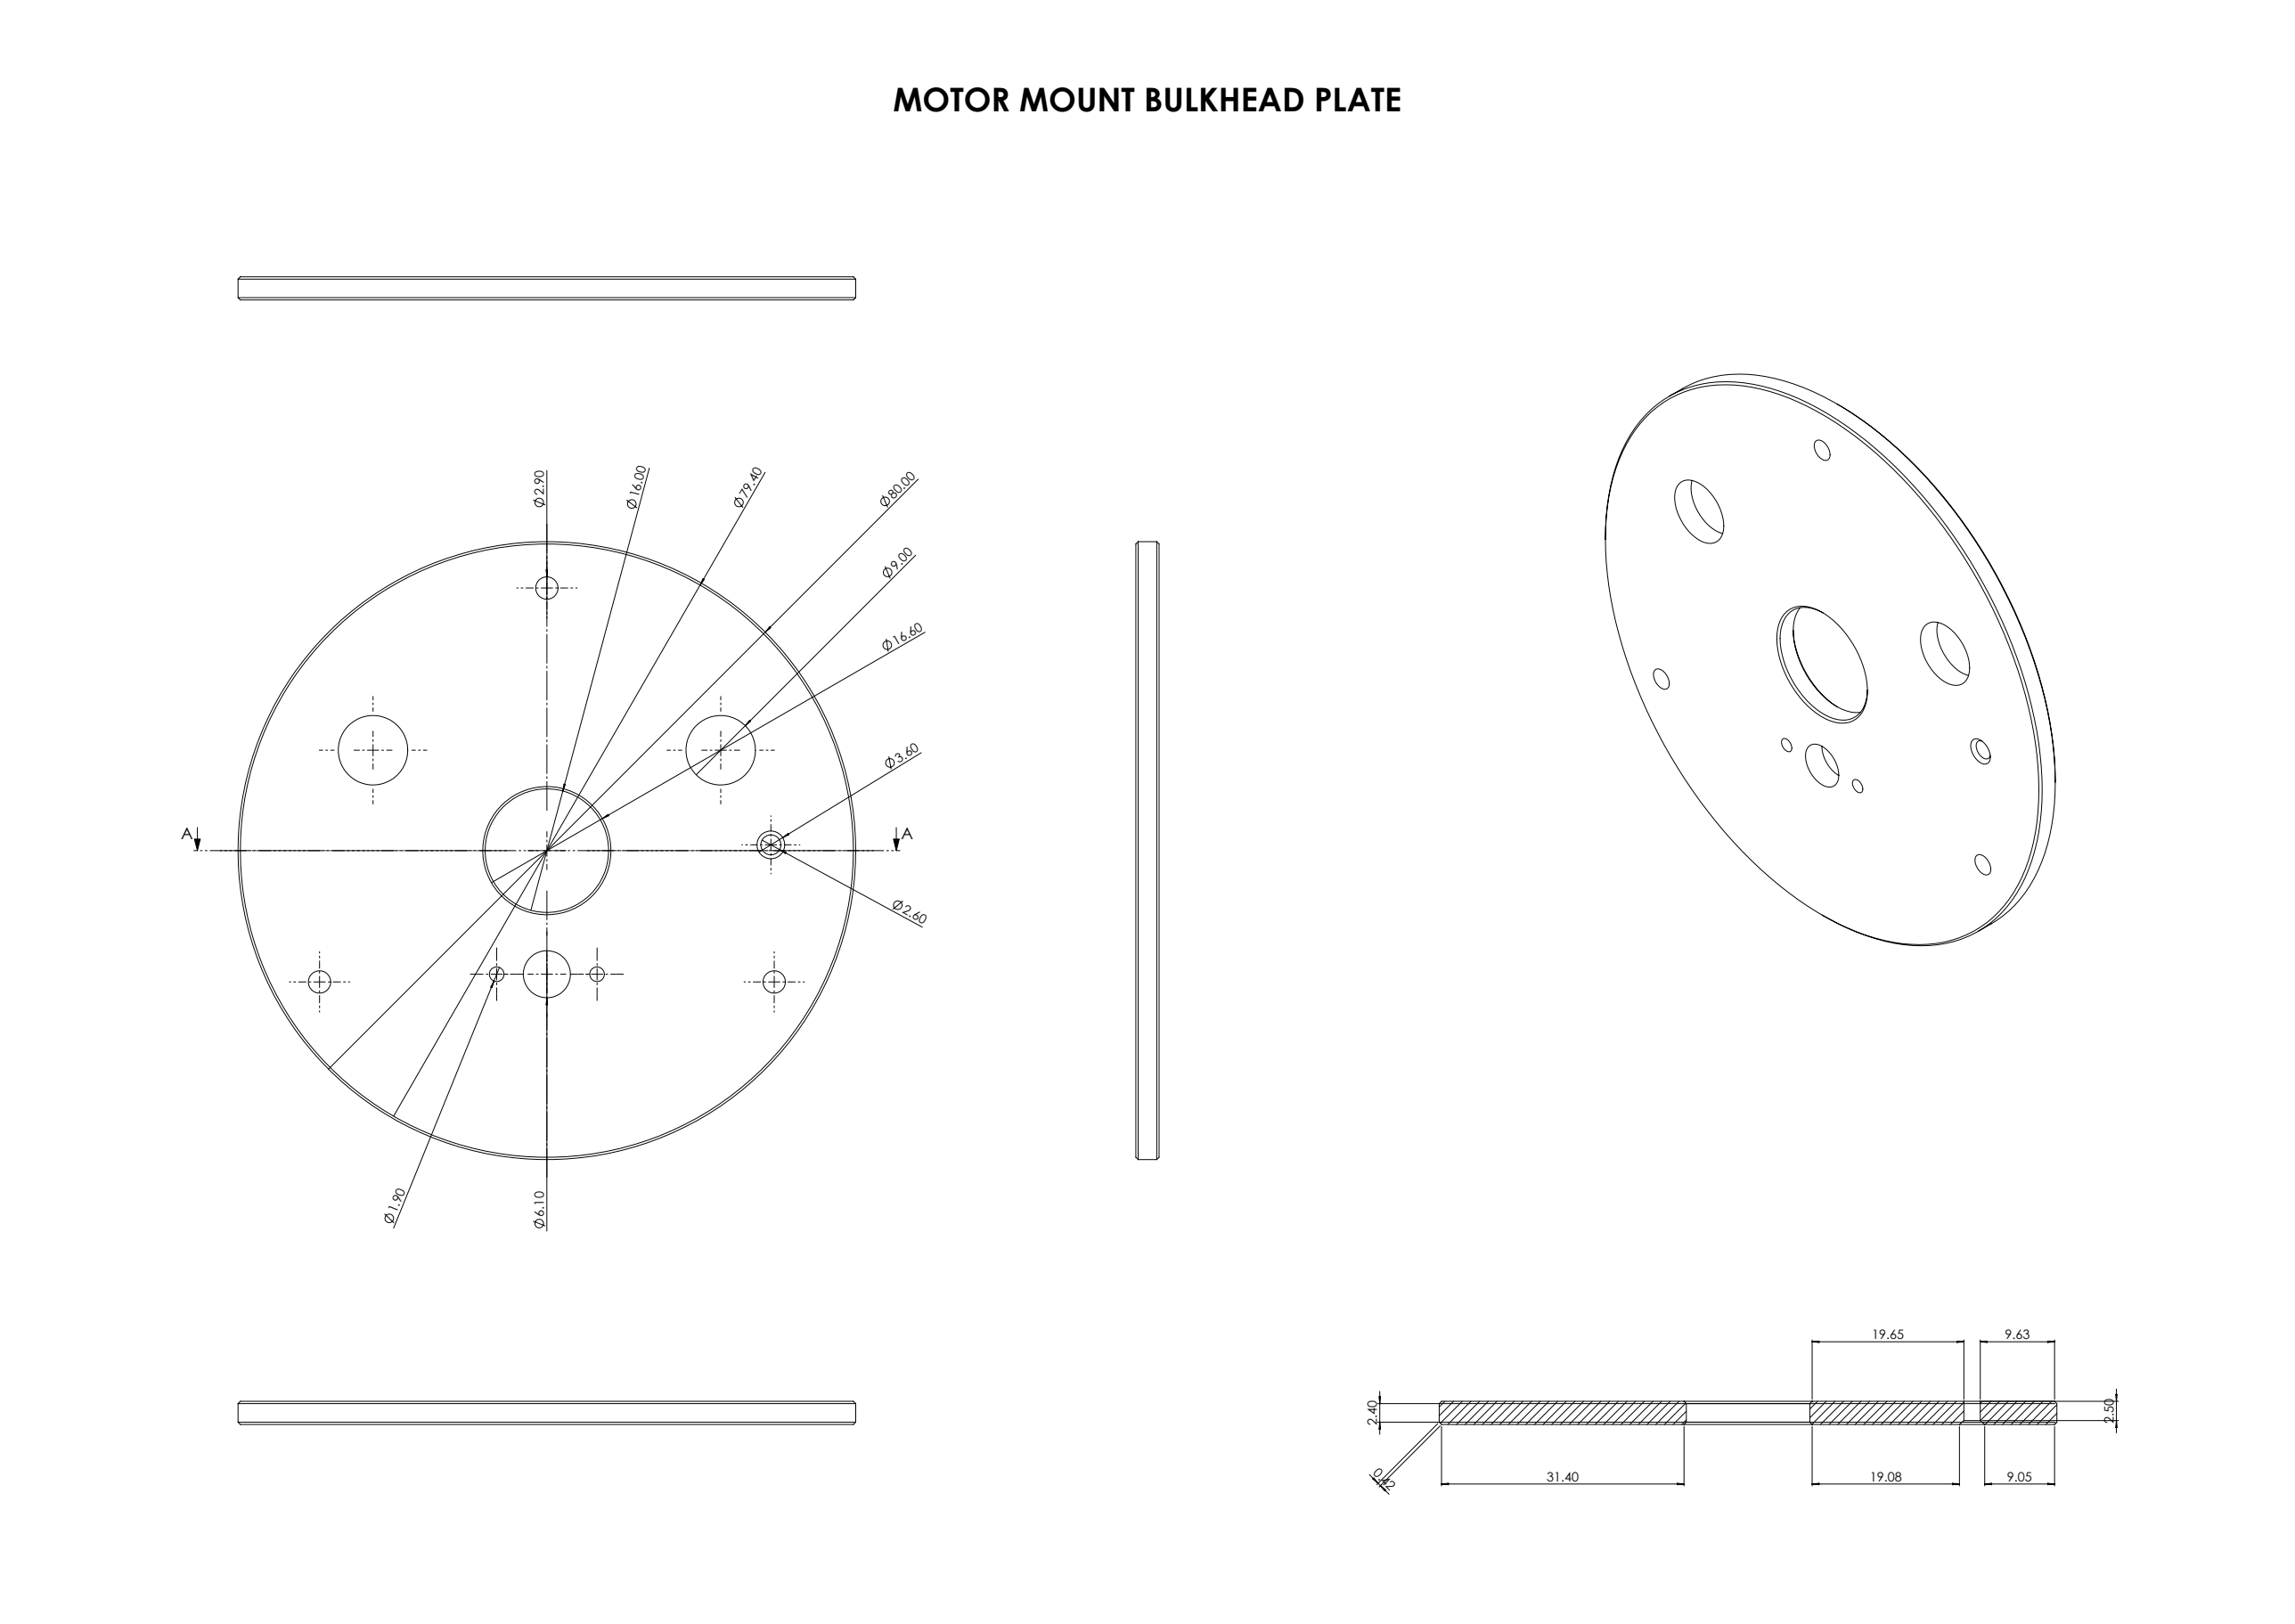
ISO-10303-21;
HEADER;
/* Generated by software containing ST-Developer
 * from STEP Tools, Inc. (www.steptools.com) 
 */

FILE_DESCRIPTION(
/* description */ (''),
/* implementation_level */ '2;1');

FILE_NAME(
/* name */ '06_Motor_Mount_Bulkhead_Plate.step',
/* time_stamp */ '2026-10-19T23:00:43-07:00',
/* author */ (''),
/* organization */ (''),
/* preprocessor_version */ 'ST-DEVELOPER v20.2',
/* originating_system */ 'Autodesk Translation Framework v15.15.0.0',
/* authorisation */ '');

FILE_SCHEMA (('AUTOMOTIVE_DESIGN { 1 0 10303 214 3 1 1 }'));
ENDSEC;

DATA;
#10=MECHANICAL_DESIGN_GEOMETRIC_PRESENTATION_REPRESENTATION('',(#1001),#55002);
#961=SHAPE_REPRESENTATION_RELATIONSHIP('SRR','None',#55109,#981);
#981=ADVANCED_BREP_SHAPE_REPRESENTATION('',(#1021),#54987);
#1001=STYLED_ITEM('',(#55372),#1021);
#1021=MANIFOLD_SOLID_BREP('Motor Mount Bulkhead',#24534);
#1169=FACE_BOUND('',#4389,.T.);
#1170=FACE_BOUND('',#4390,.T.);
#1171=FACE_BOUND('',#4391,.T.);
#1172=FACE_BOUND('',#4392,.T.);
#1173=FACE_BOUND('',#4393,.T.);
#1174=FACE_BOUND('',#4394,.T.);
#1175=FACE_BOUND('',#4395,.T.);
#1176=FACE_BOUND('',#4396,.T.);
#1177=FACE_BOUND('',#4397,.T.);
#1178=FACE_BOUND('',#4398,.T.);
#1179=FACE_BOUND('',#4401,.T.);
#1180=FACE_BOUND('',#4402,.T.);
#1181=FACE_BOUND('',#4403,.T.);
#1182=FACE_BOUND('',#4404,.T.);
#1183=FACE_BOUND('',#4405,.T.);
#1184=FACE_BOUND('',#4406,.T.);
#1185=FACE_BOUND('',#4407,.T.);
#1186=FACE_BOUND('',#4408,.T.);
#1187=FACE_BOUND('',#4409,.T.);
#1188=FACE_BOUND('',#4410,.T.);
#1423=PLANE('',#25786);
#1424=PLANE('',#25790);
#2128=CYLINDRICAL_SURFACE('',#25750,0.45);
#2129=CYLINDRICAL_SURFACE('',#25753,0.45);
#2130=CYLINDRICAL_SURFACE('',#25756,0.13);
#2131=CYLINDRICAL_SURFACE('',#25761,0.145);
#2132=CYLINDRICAL_SURFACE('',#25764,0.145);
#2133=CYLINDRICAL_SURFACE('',#25767,0.145);
#2134=CYLINDRICAL_SURFACE('',#25770,0.0950000000000001);
#2135=CYLINDRICAL_SURFACE('',#25773,0.095);
#2136=CYLINDRICAL_SURFACE('',#25776,0.305);
#2137=CYLINDRICAL_SURFACE('',#25783,0.8);
#2138=CYLINDRICAL_SURFACE('',#25795,4.);
#2879=FACE_OUTER_BOUND('',#4376,.T.);
#2880=FACE_OUTER_BOUND('',#4377,.T.);
#2881=FACE_OUTER_BOUND('',#4378,.T.);
#2882=FACE_OUTER_BOUND('',#4379,.T.);
#2883=FACE_OUTER_BOUND('',#4380,.T.);
#2884=FACE_OUTER_BOUND('',#4381,.T.);
#2885=FACE_OUTER_BOUND('',#4382,.T.);
#2886=FACE_OUTER_BOUND('',#4383,.T.);
#2887=FACE_OUTER_BOUND('',#4384,.T.);
#2888=FACE_OUTER_BOUND('',#4385,.T.);
#2889=FACE_OUTER_BOUND('',#4386,.T.);
#2890=FACE_OUTER_BOUND('',#4387,.T.);
#2891=FACE_OUTER_BOUND('',#4388,.T.);
#2892=FACE_OUTER_BOUND('',#4399,.T.);
#2893=FACE_OUTER_BOUND('',#4400,.T.);
#2894=FACE_OUTER_BOUND('',#4411,.T.);
#2895=FACE_OUTER_BOUND('',#4412,.T.);
#2896=FACE_OUTER_BOUND('',#4413,.T.);
#4376=EDGE_LOOP('',(#18006,#18007,#18008,#18009));
#4377=EDGE_LOOP('',(#18010,#18011,#18012,#18013));
#4378=EDGE_LOOP('',(#18014,#18015,#18016,#18017));
#4379=EDGE_LOOP('',(#18018,#18019,#18020,#18021));
#4380=EDGE_LOOP('',(#18022,#18023,#18024,#18025));
#4381=EDGE_LOOP('',(#18026,#18027,#18028,#18029));
#4382=EDGE_LOOP('',(#18030,#18031,#18032,#18033));
#4383=EDGE_LOOP('',(#18034,#18035,#18036,#18037));
#4384=EDGE_LOOP('',(#18038,#18039,#18040,#18041));
#4385=EDGE_LOOP('',(#18042,#18043,#18044,#18045));
#4386=EDGE_LOOP('',(#18046,#18047,#18048,#18049,#18050));
#4387=EDGE_LOOP('',(#18051,#18052,#18053,#18054,#18055,#18056));
#4388=EDGE_LOOP('',(#18057));
#4389=EDGE_LOOP('',(#18058));
#4390=EDGE_LOOP('',(#18059));
#4391=EDGE_LOOP('',(#18060));
#4392=EDGE_LOOP('',(#18061));
#4393=EDGE_LOOP('',(#18062));
#4394=EDGE_LOOP('',(#18063));
#4395=EDGE_LOOP('',(#18064));
#4396=EDGE_LOOP('',(#18065));
#4397=EDGE_LOOP('',(#18066));
#4398=EDGE_LOOP('',(#18067));
#4399=EDGE_LOOP('',(#18068,#18069,#18070,#18071,#18072));
#4400=EDGE_LOOP('',(#18073));
#4401=EDGE_LOOP('',(#18074));
#4402=EDGE_LOOP('',(#18075));
#4403=EDGE_LOOP('',(#18076));
#4404=EDGE_LOOP('',(#18077));
#4405=EDGE_LOOP('',(#18078));
#4406=EDGE_LOOP('',(#18079));
#4407=EDGE_LOOP('',(#18080));
#4408=EDGE_LOOP('',(#18081));
#4409=EDGE_LOOP('',(#18082));
#4410=EDGE_LOOP('',(#18083));
#4411=EDGE_LOOP('',(#18084,#18085,#18086,#18087,#18088));
#4412=EDGE_LOOP('',(#18089,#18090,#18091,#18092,#18093,#18094));
#4413=EDGE_LOOP('',(#18095,#18096,#18097,#18098,#18099));
#5932=LINE('',#36111,#7753);
#5933=LINE('',#36117,#7754);
#5934=LINE('',#36123,#7755);
#5935=LINE('',#36127,#7756);
#5936=LINE('',#36133,#7757);
#5937=LINE('',#36139,#7758);
#5938=LINE('',#36145,#7759);
#5939=LINE('',#36151,#7760);
#5940=LINE('',#36157,#7761);
#5941=LINE('',#36163,#7762);
#5942=LINE('',#36169,#7763);
#5943=LINE('',#36178,#7764);
#5944=LINE('',#36184,#7765);
#5945=LINE('',#36191,#7766);
#5946=LINE('',#36197,#7767);
#5947=LINE('',#36202,#7768);
#7753=VECTOR('',#29712,0.45);
#7754=VECTOR('',#29719,0.45);
#7755=VECTOR('',#29726,0.13);
#7756=VECTOR('',#29731,0.18);
#7757=VECTOR('',#29738,0.145);
#7758=VECTOR('',#29745,0.145);
#7759=VECTOR('',#29752,0.145);
#7760=VECTOR('',#29759,0.0950000000000001);
#7761=VECTOR('',#29766,0.095);
#7762=VECTOR('',#29773,0.305);
#7763=VECTOR('',#29780,0.815);
#7764=VECTOR('',#29791,0.8);
#7765=VECTOR('',#29798,0.815);
#7766=VECTOR('',#29807,3.985);
#7767=VECTOR('',#29814,4.);
#7768=VECTOR('',#29821,3.985);
#9528=CIRCLE('',#25751,0.45);
#9529=CIRCLE('',#25752,0.45);
#9530=CIRCLE('',#25754,0.45);
#9531=CIRCLE('',#25755,0.45);
#9532=CIRCLE('',#25757,0.13);
#9533=CIRCLE('',#25758,0.13);
#9534=CIRCLE('',#25760,0.18);
#9535=CIRCLE('',#25762,0.145);
#9536=CIRCLE('',#25763,0.145);
#9537=CIRCLE('',#25765,0.145);
#9538=CIRCLE('',#25766,0.145);
#9539=CIRCLE('',#25768,0.145);
#9540=CIRCLE('',#25769,0.145);
#9541=CIRCLE('',#25771,0.0950000000000001);
#9542=CIRCLE('',#25772,0.0950000000000001);
#9543=CIRCLE('',#25774,0.095);
#9544=CIRCLE('',#25775,0.095);
#9545=CIRCLE('',#25777,0.305);
#9546=CIRCLE('',#25778,0.305);
#9547=CIRCLE('',#25780,0.83);
#9548=CIRCLE('',#25781,0.8);
#9549=CIRCLE('',#25782,0.8);
#9550=CIRCLE('',#25784,0.8);
#9551=CIRCLE('',#25785,0.8);
#9552=CIRCLE('',#25787,3.97);
#9553=CIRCLE('',#25789,0.83);
#9554=CIRCLE('',#25791,3.97);
#9555=CIRCLE('',#25793,4.);
#9556=CIRCLE('',#25794,4.);
#9557=CIRCLE('',#25796,4.);
#9558=CIRCLE('',#25797,4.);
#10712=VERTEX_POINT('',#36108);
#10713=VERTEX_POINT('',#36110);
#10714=VERTEX_POINT('',#36114);
#10715=VERTEX_POINT('',#36116);
#10716=VERTEX_POINT('',#36120);
#10717=VERTEX_POINT('',#36122);
#10718=VERTEX_POINT('',#36126);
#10719=VERTEX_POINT('',#36130);
#10720=VERTEX_POINT('',#36132);
#10721=VERTEX_POINT('',#36136);
#10722=VERTEX_POINT('',#36138);
#10723=VERTEX_POINT('',#36142);
#10724=VERTEX_POINT('',#36144);
#10725=VERTEX_POINT('',#36148);
#10726=VERTEX_POINT('',#36150);
#10727=VERTEX_POINT('',#36154);
#10728=VERTEX_POINT('',#36156);
#10729=VERTEX_POINT('',#36160);
#10730=VERTEX_POINT('',#36162);
#10731=VERTEX_POINT('',#36166);
#10732=VERTEX_POINT('',#36168);
#10733=VERTEX_POINT('',#36170);
#10734=VERTEX_POINT('',#36174);
#10735=VERTEX_POINT('',#36175);
#10736=VERTEX_POINT('',#36180);
#10737=VERTEX_POINT('',#36183);
#10738=VERTEX_POINT('',#36187);
#10739=VERTEX_POINT('',#36190);
#10740=VERTEX_POINT('',#36192);
#10741=VERTEX_POINT('',#36196);
#10742=VERTEX_POINT('',#36198);
#13411=EDGE_CURVE('',#10712,#10712,#9528,.T.);
#13412=EDGE_CURVE('',#10712,#10713,#5932,.T.);
#13413=EDGE_CURVE('',#10713,#10713,#9529,.T.);
#13414=EDGE_CURVE('',#10714,#10714,#9530,.T.);
#13415=EDGE_CURVE('',#10714,#10715,#5933,.T.);
#13416=EDGE_CURVE('',#10715,#10715,#9531,.T.);
#13417=EDGE_CURVE('',#10716,#10716,#9532,.T.);
#13418=EDGE_CURVE('',#10716,#10717,#5934,.T.);
#13419=EDGE_CURVE('',#10717,#10717,#9533,.T.);
#13420=EDGE_CURVE('',#10717,#10718,#5935,.T.);
#13421=EDGE_CURVE('',#10718,#10718,#9534,.T.);
#13422=EDGE_CURVE('',#10719,#10719,#9535,.T.);
#13423=EDGE_CURVE('',#10719,#10720,#5936,.T.);
#13424=EDGE_CURVE('',#10720,#10720,#9536,.T.);
#13425=EDGE_CURVE('',#10721,#10721,#9537,.T.);
#13426=EDGE_CURVE('',#10721,#10722,#5937,.T.);
#13427=EDGE_CURVE('',#10722,#10722,#9538,.T.);
#13428=EDGE_CURVE('',#10723,#10723,#9539,.T.);
#13429=EDGE_CURVE('',#10723,#10724,#5938,.T.);
#13430=EDGE_CURVE('',#10724,#10724,#9540,.T.);
#13431=EDGE_CURVE('',#10725,#10725,#9541,.T.);
#13432=EDGE_CURVE('',#10725,#10726,#5939,.T.);
#13433=EDGE_CURVE('',#10726,#10726,#9542,.T.);
#13434=EDGE_CURVE('',#10727,#10727,#9543,.T.);
#13435=EDGE_CURVE('',#10727,#10728,#5940,.T.);
#13436=EDGE_CURVE('',#10728,#10728,#9544,.T.);
#13437=EDGE_CURVE('',#10729,#10729,#9545,.T.);
#13438=EDGE_CURVE('',#10729,#10730,#5941,.T.);
#13439=EDGE_CURVE('',#10730,#10730,#9546,.T.);
#13440=EDGE_CURVE('',#10731,#10731,#9547,.T.);
#13441=EDGE_CURVE('',#10731,#10732,#5942,.T.);
#13442=EDGE_CURVE('',#10732,#10733,#9548,.T.);
#13443=EDGE_CURVE('',#10733,#10732,#9549,.T.);
#13444=EDGE_CURVE('',#10734,#10735,#9550,.T.);
#13445=EDGE_CURVE('',#10735,#10734,#9551,.T.);
#13446=EDGE_CURVE('',#10735,#10733,#5943,.T.);
#13447=EDGE_CURVE('',#10736,#10736,#9552,.T.);
#13448=EDGE_CURVE('',#10734,#10737,#5944,.T.);
#13449=EDGE_CURVE('',#10737,#10737,#9553,.T.);
#13450=EDGE_CURVE('',#10738,#10738,#9554,.T.);
#13451=EDGE_CURVE('',#10738,#10739,#5945,.T.);
#13452=EDGE_CURVE('',#10739,#10740,#9555,.T.);
#13453=EDGE_CURVE('',#10740,#10739,#9556,.T.);
#13454=EDGE_CURVE('',#10740,#10741,#5946,.T.);
#13455=EDGE_CURVE('',#10742,#10741,#9557,.T.);
#13456=EDGE_CURVE('',#10741,#10742,#9558,.T.);
#13457=EDGE_CURVE('',#10742,#10736,#5947,.T.);
#18006=ORIENTED_EDGE('',*,*,#13411,.F.);
#18007=ORIENTED_EDGE('',*,*,#13412,.T.);
#18008=ORIENTED_EDGE('',*,*,#13413,.F.);
#18009=ORIENTED_EDGE('',*,*,#13412,.F.);
#18010=ORIENTED_EDGE('',*,*,#13414,.F.);
#18011=ORIENTED_EDGE('',*,*,#13415,.T.);
#18012=ORIENTED_EDGE('',*,*,#13416,.F.);
#18013=ORIENTED_EDGE('',*,*,#13415,.F.);
#18014=ORIENTED_EDGE('',*,*,#13417,.F.);
#18015=ORIENTED_EDGE('',*,*,#13418,.T.);
#18016=ORIENTED_EDGE('',*,*,#13419,.T.);
#18017=ORIENTED_EDGE('',*,*,#13418,.F.);
#18018=ORIENTED_EDGE('',*,*,#13419,.F.);
#18019=ORIENTED_EDGE('',*,*,#13420,.T.);
#18020=ORIENTED_EDGE('',*,*,#13421,.F.);
#18021=ORIENTED_EDGE('',*,*,#13420,.F.);
#18022=ORIENTED_EDGE('',*,*,#13422,.F.);
#18023=ORIENTED_EDGE('',*,*,#13423,.T.);
#18024=ORIENTED_EDGE('',*,*,#13424,.F.);
#18025=ORIENTED_EDGE('',*,*,#13423,.F.);
#18026=ORIENTED_EDGE('',*,*,#13425,.F.);
#18027=ORIENTED_EDGE('',*,*,#13426,.T.);
#18028=ORIENTED_EDGE('',*,*,#13427,.F.);
#18029=ORIENTED_EDGE('',*,*,#13426,.F.);
#18030=ORIENTED_EDGE('',*,*,#13428,.F.);
#18031=ORIENTED_EDGE('',*,*,#13429,.T.);
#18032=ORIENTED_EDGE('',*,*,#13430,.F.);
#18033=ORIENTED_EDGE('',*,*,#13429,.F.);
#18034=ORIENTED_EDGE('',*,*,#13431,.F.);
#18035=ORIENTED_EDGE('',*,*,#13432,.T.);
#18036=ORIENTED_EDGE('',*,*,#13433,.F.);
#18037=ORIENTED_EDGE('',*,*,#13432,.F.);
#18038=ORIENTED_EDGE('',*,*,#13434,.F.);
#18039=ORIENTED_EDGE('',*,*,#13435,.T.);
#18040=ORIENTED_EDGE('',*,*,#13436,.F.);
#18041=ORIENTED_EDGE('',*,*,#13435,.F.);
#18042=ORIENTED_EDGE('',*,*,#13437,.F.);
#18043=ORIENTED_EDGE('',*,*,#13438,.T.);
#18044=ORIENTED_EDGE('',*,*,#13439,.F.);
#18045=ORIENTED_EDGE('',*,*,#13438,.F.);
#18046=ORIENTED_EDGE('',*,*,#13440,.T.);
#18047=ORIENTED_EDGE('',*,*,#13441,.T.);
#18048=ORIENTED_EDGE('',*,*,#13442,.T.);
#18049=ORIENTED_EDGE('',*,*,#13443,.T.);
#18050=ORIENTED_EDGE('',*,*,#13441,.F.);
#18051=ORIENTED_EDGE('',*,*,#13444,.F.);
#18052=ORIENTED_EDGE('',*,*,#13445,.F.);
#18053=ORIENTED_EDGE('',*,*,#13446,.T.);
#18054=ORIENTED_EDGE('',*,*,#13442,.F.);
#18055=ORIENTED_EDGE('',*,*,#13443,.F.);
#18056=ORIENTED_EDGE('',*,*,#13446,.F.);
#18057=ORIENTED_EDGE('',*,*,#13447,.F.);
#18058=ORIENTED_EDGE('',*,*,#13414,.T.);
#18059=ORIENTED_EDGE('',*,*,#13440,.F.);
#18060=ORIENTED_EDGE('',*,*,#13437,.T.);
#18061=ORIENTED_EDGE('',*,*,#13434,.T.);
#18062=ORIENTED_EDGE('',*,*,#13431,.T.);
#18063=ORIENTED_EDGE('',*,*,#13428,.T.);
#18064=ORIENTED_EDGE('',*,*,#13425,.T.);
#18065=ORIENTED_EDGE('',*,*,#13422,.T.);
#18066=ORIENTED_EDGE('',*,*,#13417,.T.);
#18067=ORIENTED_EDGE('',*,*,#13411,.T.);
#18068=ORIENTED_EDGE('',*,*,#13444,.T.);
#18069=ORIENTED_EDGE('',*,*,#13445,.T.);
#18070=ORIENTED_EDGE('',*,*,#13448,.T.);
#18071=ORIENTED_EDGE('',*,*,#13449,.T.);
#18072=ORIENTED_EDGE('',*,*,#13448,.F.);
#18073=ORIENTED_EDGE('',*,*,#13450,.F.);
#18074=ORIENTED_EDGE('',*,*,#13416,.T.);
#18075=ORIENTED_EDGE('',*,*,#13449,.F.);
#18076=ORIENTED_EDGE('',*,*,#13439,.T.);
#18077=ORIENTED_EDGE('',*,*,#13436,.T.);
#18078=ORIENTED_EDGE('',*,*,#13433,.T.);
#18079=ORIENTED_EDGE('',*,*,#13430,.T.);
#18080=ORIENTED_EDGE('',*,*,#13427,.T.);
#18081=ORIENTED_EDGE('',*,*,#13424,.T.);
#18082=ORIENTED_EDGE('',*,*,#13421,.T.);
#18083=ORIENTED_EDGE('',*,*,#13413,.T.);
#18084=ORIENTED_EDGE('',*,*,#13450,.T.);
#18085=ORIENTED_EDGE('',*,*,#13451,.T.);
#18086=ORIENTED_EDGE('',*,*,#13452,.T.);
#18087=ORIENTED_EDGE('',*,*,#13453,.T.);
#18088=ORIENTED_EDGE('',*,*,#13451,.F.);
#18089=ORIENTED_EDGE('',*,*,#13452,.F.);
#18090=ORIENTED_EDGE('',*,*,#13453,.F.);
#18091=ORIENTED_EDGE('',*,*,#13454,.T.);
#18092=ORIENTED_EDGE('',*,*,#13455,.F.);
#18093=ORIENTED_EDGE('',*,*,#13456,.F.);
#18094=ORIENTED_EDGE('',*,*,#13454,.F.);
#18095=ORIENTED_EDGE('',*,*,#13455,.T.);
#18096=ORIENTED_EDGE('',*,*,#13456,.T.);
#18097=ORIENTED_EDGE('',*,*,#13457,.T.);
#18098=ORIENTED_EDGE('',*,*,#13447,.T.);
#18099=ORIENTED_EDGE('',*,*,#13457,.F.);
#23098=CONICAL_SURFACE('',#25759,0.18,0.785398163397448);
#23099=CONICAL_SURFACE('',#25779,0.815,0.785398163397459);
#23100=CONICAL_SURFACE('',#25788,0.815,0.785398163397459);
#23101=CONICAL_SURFACE('',#25792,3.985,0.785398163397456);
#23102=CONICAL_SURFACE('',#25798,3.985,0.785398163397456);
#23632=ADVANCED_FACE('',(#2879),#2128,.F.);
#23633=ADVANCED_FACE('',(#2880),#2129,.F.);
#23634=ADVANCED_FACE('',(#2881),#2130,.F.);
#23635=ADVANCED_FACE('',(#2882),#23098,.F.);
#23636=ADVANCED_FACE('',(#2883),#2131,.F.);
#23637=ADVANCED_FACE('',(#2884),#2132,.F.);
#23638=ADVANCED_FACE('',(#2885),#2133,.F.);
#23639=ADVANCED_FACE('',(#2886),#2134,.F.);
#23640=ADVANCED_FACE('',(#2887),#2135,.F.);
#23641=ADVANCED_FACE('',(#2888),#2136,.F.);
#23642=ADVANCED_FACE('',(#2889),#23099,.F.);
#23643=ADVANCED_FACE('',(#2890),#2137,.F.);
#23644=ADVANCED_FACE('',(#2891,#1169,#1170,#1171,#1172,#1173,#1174,#1175,
#1176,#1177,#1178),#1423,.T.);
#23645=ADVANCED_FACE('',(#2892),#23100,.F.);
#23646=ADVANCED_FACE('',(#2893,#1179,#1180,#1181,#1182,#1183,#1184,#1185,
#1186,#1187,#1188),#1424,.T.);
#23647=ADVANCED_FACE('',(#2894),#23101,.T.);
#23648=ADVANCED_FACE('',(#2895),#2138,.T.);
#23649=ADVANCED_FACE('',(#2896),#23102,.T.);
#24534=CLOSED_SHELL('',(#23632,#23633,#23634,#23635,#23636,#23637,#23638,
#23639,#23640,#23641,#23642,#23643,#23644,#23645,#23646,#23647,#23648,#23649));
#25749=AXIS2_PLACEMENT_3D('',#36106,#29706,#29707);
#25750=AXIS2_PLACEMENT_3D('',#36107,#29708,#29709);
#25751=AXIS2_PLACEMENT_3D('',#36109,#29710,#29711);
#25752=AXIS2_PLACEMENT_3D('',#36112,#29713,#29714);
#25753=AXIS2_PLACEMENT_3D('',#36113,#29715,#29716);
#25754=AXIS2_PLACEMENT_3D('',#36115,#29717,#29718);
#25755=AXIS2_PLACEMENT_3D('',#36118,#29720,#29721);
#25756=AXIS2_PLACEMENT_3D('',#36119,#29722,#29723);
#25757=AXIS2_PLACEMENT_3D('',#36121,#29724,#29725);
#25758=AXIS2_PLACEMENT_3D('',#36124,#29727,#29728);
#25759=AXIS2_PLACEMENT_3D('',#36125,#29729,#29730);
#25760=AXIS2_PLACEMENT_3D('',#36128,#29732,#29733);
#25761=AXIS2_PLACEMENT_3D('',#36129,#29734,#29735);
#25762=AXIS2_PLACEMENT_3D('',#36131,#29736,#29737);
#25763=AXIS2_PLACEMENT_3D('',#36134,#29739,#29740);
#25764=AXIS2_PLACEMENT_3D('',#36135,#29741,#29742);
#25765=AXIS2_PLACEMENT_3D('',#36137,#29743,#29744);
#25766=AXIS2_PLACEMENT_3D('',#36140,#29746,#29747);
#25767=AXIS2_PLACEMENT_3D('',#36141,#29748,#29749);
#25768=AXIS2_PLACEMENT_3D('',#36143,#29750,#29751);
#25769=AXIS2_PLACEMENT_3D('',#36146,#29753,#29754);
#25770=AXIS2_PLACEMENT_3D('',#36147,#29755,#29756);
#25771=AXIS2_PLACEMENT_3D('',#36149,#29757,#29758);
#25772=AXIS2_PLACEMENT_3D('',#36152,#29760,#29761);
#25773=AXIS2_PLACEMENT_3D('',#36153,#29762,#29763);
#25774=AXIS2_PLACEMENT_3D('',#36155,#29764,#29765);
#25775=AXIS2_PLACEMENT_3D('',#36158,#29767,#29768);
#25776=AXIS2_PLACEMENT_3D('',#36159,#29769,#29770);
#25777=AXIS2_PLACEMENT_3D('',#36161,#29771,#29772);
#25778=AXIS2_PLACEMENT_3D('',#36164,#29774,#29775);
#25779=AXIS2_PLACEMENT_3D('',#36165,#29776,#29777);
#25780=AXIS2_PLACEMENT_3D('',#36167,#29778,#29779);
#25781=AXIS2_PLACEMENT_3D('',#36171,#29781,#29782);
#25782=AXIS2_PLACEMENT_3D('',#36172,#29783,#29784);
#25783=AXIS2_PLACEMENT_3D('',#36173,#29785,#29786);
#25784=AXIS2_PLACEMENT_3D('',#36176,#29787,#29788);
#25785=AXIS2_PLACEMENT_3D('',#36177,#29789,#29790);
#25786=AXIS2_PLACEMENT_3D('',#36179,#29792,#29793);
#25787=AXIS2_PLACEMENT_3D('',#36181,#29794,#29795);
#25788=AXIS2_PLACEMENT_3D('',#36182,#29796,#29797);
#25789=AXIS2_PLACEMENT_3D('',#36185,#29799,#29800);
#25790=AXIS2_PLACEMENT_3D('',#36186,#29801,#29802);
#25791=AXIS2_PLACEMENT_3D('',#36188,#29803,#29804);
#25792=AXIS2_PLACEMENT_3D('',#36189,#29805,#29806);
#25793=AXIS2_PLACEMENT_3D('',#36193,#29808,#29809);
#25794=AXIS2_PLACEMENT_3D('',#36194,#29810,#29811);
#25795=AXIS2_PLACEMENT_3D('',#36195,#29812,#29813);
#25796=AXIS2_PLACEMENT_3D('',#36199,#29815,#29816);
#25797=AXIS2_PLACEMENT_3D('',#36200,#29817,#29818);
#25798=AXIS2_PLACEMENT_3D('',#36201,#29819,#29820);
#29706=DIRECTION('axis',(0.,0.,1.));
#29707=DIRECTION('refdir',(1.,0.,0.));
#29708=DIRECTION('center_axis',(0.,0.,1.));
#29709=DIRECTION('ref_axis',(1.,0.,0.));
#29710=DIRECTION('center_axis',(0.,0.,1.));
#29711=DIRECTION('ref_axis',(1.,0.,0.));
#29712=DIRECTION('',(0.,0.,1.));
#29713=DIRECTION('center_axis',(0.,0.,-1.));
#29714=DIRECTION('ref_axis',(1.,0.,0.));
#29715=DIRECTION('center_axis',(0.,0.,1.));
#29716=DIRECTION('ref_axis',(1.,0.,0.));
#29717=DIRECTION('center_axis',(0.,0.,1.));
#29718=DIRECTION('ref_axis',(1.,0.,0.));
#29719=DIRECTION('',(0.,0.,1.));
#29720=DIRECTION('center_axis',(0.,0.,-1.));
#29721=DIRECTION('ref_axis',(1.,0.,0.));
#29722=DIRECTION('center_axis',(0.,0.,1.));
#29723=DIRECTION('ref_axis',(1.,0.,0.));
#29724=DIRECTION('center_axis',(0.,0.,1.));
#29725=DIRECTION('ref_axis',(1.,0.,0.));
#29726=DIRECTION('',(0.,0.,1.));
#29727=DIRECTION('center_axis',(0.,0.,1.));
#29728=DIRECTION('ref_axis',(1.,0.,0.));
#29729=DIRECTION('center_axis',(0.,0.,1.));
#29730=DIRECTION('ref_axis',(1.,0.,0.));
#29731=DIRECTION('',(-0.707106781186548,-8.65956056235493E-17,0.707106781186548));
#29732=DIRECTION('center_axis',(0.,0.,-1.));
#29733=DIRECTION('ref_axis',(1.,0.,0.));
#29734=DIRECTION('center_axis',(0.,0.,1.));
#29735=DIRECTION('ref_axis',(1.,0.,0.));
#29736=DIRECTION('center_axis',(0.,0.,1.));
#29737=DIRECTION('ref_axis',(1.,0.,0.));
#29738=DIRECTION('',(0.,0.,1.));
#29739=DIRECTION('center_axis',(0.,0.,-1.));
#29740=DIRECTION('ref_axis',(1.,0.,0.));
#29741=DIRECTION('center_axis',(0.,0.,1.));
#29742=DIRECTION('ref_axis',(1.,0.,0.));
#29743=DIRECTION('center_axis',(0.,0.,1.));
#29744=DIRECTION('ref_axis',(1.,0.,0.));
#29745=DIRECTION('',(0.,0.,1.));
#29746=DIRECTION('center_axis',(0.,0.,-1.));
#29747=DIRECTION('ref_axis',(1.,0.,0.));
#29748=DIRECTION('center_axis',(0.,0.,1.));
#29749=DIRECTION('ref_axis',(1.,0.,0.));
#29750=DIRECTION('center_axis',(0.,0.,1.));
#29751=DIRECTION('ref_axis',(1.,0.,0.));
#29752=DIRECTION('',(0.,0.,1.));
#29753=DIRECTION('center_axis',(0.,0.,-1.));
#29754=DIRECTION('ref_axis',(1.,0.,0.));
#29755=DIRECTION('center_axis',(0.,0.,1.));
#29756=DIRECTION('ref_axis',(1.,0.,0.));
#29757=DIRECTION('center_axis',(0.,0.,1.));
#29758=DIRECTION('ref_axis',(1.,0.,0.));
#29759=DIRECTION('',(0.,0.,1.));
#29760=DIRECTION('center_axis',(0.,0.,-1.));
#29761=DIRECTION('ref_axis',(1.,0.,0.));
#29762=DIRECTION('center_axis',(0.,0.,1.));
#29763=DIRECTION('ref_axis',(1.,0.,0.));
#29764=DIRECTION('center_axis',(0.,0.,1.));
#29765=DIRECTION('ref_axis',(1.,0.,0.));
#29766=DIRECTION('',(0.,0.,1.));
#29767=DIRECTION('center_axis',(0.,0.,-1.));
#29768=DIRECTION('ref_axis',(1.,0.,0.));
#29769=DIRECTION('center_axis',(0.,0.,1.));
#29770=DIRECTION('ref_axis',(1.,0.,0.));
#29771=DIRECTION('center_axis',(0.,0.,1.));
#29772=DIRECTION('ref_axis',(1.,0.,0.));
#29773=DIRECTION('',(0.,0.,1.));
#29774=DIRECTION('center_axis',(0.,0.,-1.));
#29775=DIRECTION('ref_axis',(1.,0.,0.));
#29776=DIRECTION('center_axis',(0.,0.,-1.));
#29777=DIRECTION('ref_axis',(-1.,0.,0.));
#29778=DIRECTION('center_axis',(0.,0.,-1.));
#29779=DIRECTION('ref_axis',(-1.,0.,0.));
#29780=DIRECTION('',(-0.707106781186555,8.65956056235503E-17,0.70710678118654));
#29781=DIRECTION('center_axis',(0.,0.,1.));
#29782=DIRECTION('ref_axis',(-1.,0.,0.));
#29783=DIRECTION('center_axis',(0.,0.,1.));
#29784=DIRECTION('ref_axis',(-1.,0.,0.));
#29785=DIRECTION('center_axis',(0.,0.,1.));
#29786=DIRECTION('ref_axis',(1.,0.,0.));
#29787=DIRECTION('center_axis',(0.,0.,-1.));
#29788=DIRECTION('ref_axis',(-1.,0.,0.));
#29789=DIRECTION('center_axis',(0.,0.,-1.));
#29790=DIRECTION('ref_axis',(-1.,0.,0.));
#29791=DIRECTION('',(0.,0.,-1.));
#29792=DIRECTION('center_axis',(0.,0.,-1.));
#29793=DIRECTION('ref_axis',(-1.,0.,0.));
#29794=DIRECTION('center_axis',(0.,0.,1.));
#29795=DIRECTION('ref_axis',(-1.,0.,0.));
#29796=DIRECTION('center_axis',(0.,0.,1.));
#29797=DIRECTION('ref_axis',(-1.,0.,0.));
#29798=DIRECTION('',(0.707106781186555,-8.65956056235503E-17,0.70710678118654));
#29799=DIRECTION('center_axis',(0.,0.,1.));
#29800=DIRECTION('ref_axis',(-1.,0.,0.));
#29801=DIRECTION('center_axis',(0.,0.,1.));
#29802=DIRECTION('ref_axis',(1.,0.,0.));
#29803=DIRECTION('center_axis',(0.,0.,-1.));
#29804=DIRECTION('ref_axis',(-1.,0.,0.));
#29805=DIRECTION('center_axis',(0.,0.,-1.));
#29806=DIRECTION('ref_axis',(-1.,0.,0.));
#29807=DIRECTION('',(0.707106781186553,8.659560562355E-17,-0.707106781186542));
#29808=DIRECTION('center_axis',(0.,0.,1.));
#29809=DIRECTION('ref_axis',(-1.,0.,0.));
#29810=DIRECTION('center_axis',(0.,0.,1.));
#29811=DIRECTION('ref_axis',(-1.,0.,0.));
#29812=DIRECTION('center_axis',(0.,0.,1.));
#29813=DIRECTION('ref_axis',(1.,0.,0.));
#29814=DIRECTION('',(0.,0.,-1.));
#29815=DIRECTION('center_axis',(0.,0.,-1.));
#29816=DIRECTION('ref_axis',(-1.,0.,0.));
#29817=DIRECTION('center_axis',(0.,0.,-1.));
#29818=DIRECTION('ref_axis',(-1.,0.,0.));
#29819=DIRECTION('center_axis',(0.,0.,1.));
#29820=DIRECTION('ref_axis',(-1.,0.,0.));
#29821=DIRECTION('',(-0.707106781186553,-8.659560562355E-17,-0.707106781186542));
#36106=CARTESIAN_POINT('',(0.,0.,0.));
#36107=CARTESIAN_POINT('Origin',(-2.25166604983954,1.3,10.25));
#36108=CARTESIAN_POINT('',(-2.70166604983954,1.3,10.1));
#36109=CARTESIAN_POINT('Origin',(-2.25166604983954,1.3,10.1));
#36110=CARTESIAN_POINT('',(-2.70166604983954,1.3,10.4));
#36111=CARTESIAN_POINT('',(-2.70166604983954,1.3,10.25));
#36112=CARTESIAN_POINT('Origin',(-2.25166604983954,1.3,10.4));
#36113=CARTESIAN_POINT('Origin',(2.25166604983954,1.3,10.25));
#36114=CARTESIAN_POINT('',(1.80166604983954,1.3,10.1));
#36115=CARTESIAN_POINT('Origin',(2.25166604983954,1.3,10.1));
#36116=CARTESIAN_POINT('',(1.80166604983954,1.3,10.4));
#36117=CARTESIAN_POINT('',(1.80166604983954,1.3,10.25));
#36118=CARTESIAN_POINT('Origin',(2.25166604983954,1.3,10.4));
#36119=CARTESIAN_POINT('Origin',(2.90118510267787,0.0750000000000004,10.215));
#36120=CARTESIAN_POINT('',(2.77118510267787,0.0750000000000003,10.1));
#36121=CARTESIAN_POINT('Origin',(2.90118510267787,0.0750000000000004,10.1));
#36122=CARTESIAN_POINT('',(2.77118510267787,0.0750000000000003,10.35));
#36123=CARTESIAN_POINT('',(2.77118510267787,0.0750000000000003,10.215));
#36124=CARTESIAN_POINT('Origin',(2.90118510267787,0.0750000000000004,10.35));
#36125=CARTESIAN_POINT('Origin',(2.90118510267787,0.0750000000000004,10.4));
#36126=CARTESIAN_POINT('',(2.72118510267787,0.0750000000000004,10.4));
#36127=CARTESIAN_POINT('',(2.72118510267787,0.0750000000000003,10.4));
#36128=CARTESIAN_POINT('Origin',(2.90118510267787,0.0750000000000004,10.4));
#36129=CARTESIAN_POINT('Origin',(2.94448637286709,-1.7,10.25));
#36130=CARTESIAN_POINT('',(2.79948637286709,-1.7,10.1));
#36131=CARTESIAN_POINT('Origin',(2.94448637286709,-1.7,10.1));
#36132=CARTESIAN_POINT('',(2.79948637286709,-1.7,10.4));
#36133=CARTESIAN_POINT('',(2.79948637286709,-1.7,10.25));
#36134=CARTESIAN_POINT('Origin',(2.94448637286709,-1.7,10.4));
#36135=CARTESIAN_POINT('Origin',(-2.94448637286709,-1.7,10.25));
#36136=CARTESIAN_POINT('',(-3.08948637286709,-1.7,10.1));
#36137=CARTESIAN_POINT('Origin',(-2.94448637286709,-1.7,10.1));
#36138=CARTESIAN_POINT('',(-3.08948637286709,-1.7,10.4));
#36139=CARTESIAN_POINT('',(-3.08948637286709,-1.7,10.25));
#36140=CARTESIAN_POINT('Origin',(-2.94448637286709,-1.7,10.4));
#36141=CARTESIAN_POINT('Origin',(2.0818995585505E-16,3.4,10.25));
#36142=CARTESIAN_POINT('',(-0.145,3.4,10.1));
#36143=CARTESIAN_POINT('Origin',(2.0818995585505E-16,3.4,10.1));
#36144=CARTESIAN_POINT('',(-0.145,3.4,10.4));
#36145=CARTESIAN_POINT('',(-0.145,3.4,10.25));
#36146=CARTESIAN_POINT('Origin',(2.0818995585505E-16,3.4,10.4));
#36147=CARTESIAN_POINT('Origin',(-0.65,-1.6,10.25));
#36148=CARTESIAN_POINT('',(-0.745,-1.6,10.1));
#36149=CARTESIAN_POINT('Origin',(-0.65,-1.6,10.1));
#36150=CARTESIAN_POINT('',(-0.745,-1.6,10.4));
#36151=CARTESIAN_POINT('',(-0.745,-1.6,10.25));
#36152=CARTESIAN_POINT('Origin',(-0.65,-1.6,10.4));
#36153=CARTESIAN_POINT('Origin',(0.65,-1.6,10.25));
#36154=CARTESIAN_POINT('',(0.555,-1.6,10.1));
#36155=CARTESIAN_POINT('Origin',(0.65,-1.6,10.1));
#36156=CARTESIAN_POINT('',(0.555,-1.6,10.4));
#36157=CARTESIAN_POINT('',(0.555,-1.6,10.25));
#36158=CARTESIAN_POINT('Origin',(0.65,-1.6,10.4));
#36159=CARTESIAN_POINT('Origin',(0.,-1.6,10.25));
#36160=CARTESIAN_POINT('',(-0.305,-1.6,10.1));
#36161=CARTESIAN_POINT('Origin',(0.,-1.6,10.1));
#36162=CARTESIAN_POINT('',(-0.305,-1.6,10.4));
#36163=CARTESIAN_POINT('',(-0.305,-1.6,10.25));
#36164=CARTESIAN_POINT('Origin',(0.,-1.6,10.4));
#36165=CARTESIAN_POINT('Origin',(0.,0.,10.115));
#36166=CARTESIAN_POINT('',(0.83,-1.0164568432923E-16,10.1));
#36167=CARTESIAN_POINT('Origin',(0.,0.,10.1));
#36168=CARTESIAN_POINT('',(0.8,9.79717439317883E-17,10.13));
#36169=CARTESIAN_POINT('',(0.815,-9.98087141305093E-17,10.115));
#36170=CARTESIAN_POINT('',(-0.8,-9.79717439317883E-17,10.13));
#36171=CARTESIAN_POINT('Origin',(0.,0.,10.13));
#36172=CARTESIAN_POINT('Origin',(0.,0.,10.13));
#36173=CARTESIAN_POINT('Origin',(0.,0.,10.25));
#36174=CARTESIAN_POINT('',(0.8,-9.79717439317883E-17,10.37));
#36175=CARTESIAN_POINT('',(-0.8,-9.79717439317883E-17,10.37));
#36176=CARTESIAN_POINT('Origin',(0.,0.,10.37));
#36177=CARTESIAN_POINT('Origin',(0.,0.,10.37));
#36178=CARTESIAN_POINT('',(-0.8,-9.79717439317883E-17,10.25));
#36179=CARTESIAN_POINT('Origin',(4.,0.,10.1));
#36180=CARTESIAN_POINT('',(3.97,4.86184779261499E-16,10.1));
#36181=CARTESIAN_POINT('Origin',(0.,0.,10.1));
#36182=CARTESIAN_POINT('Origin',(0.,0.,10.385));
#36183=CARTESIAN_POINT('',(0.83,1.0164568432923E-16,10.4));
#36184=CARTESIAN_POINT('',(0.815,-9.98087141305093E-17,10.385));
#36185=CARTESIAN_POINT('Origin',(0.,0.,10.4));
#36186=CARTESIAN_POINT('Origin',(0.8,0.,10.4));
#36187=CARTESIAN_POINT('',(3.97,-4.86184779261499E-16,10.4));
#36188=CARTESIAN_POINT('Origin',(0.,0.,10.4));
#36189=CARTESIAN_POINT('Origin',(0.,0.,10.385));
#36190=CARTESIAN_POINT('',(4.,4.89858719658941E-16,10.37));
#36191=CARTESIAN_POINT('',(3.985,4.8802174946022E-16,10.385));
#36192=CARTESIAN_POINT('',(-4.,-4.89858719658941E-16,10.37));
#36193=CARTESIAN_POINT('Origin',(0.,0.,10.37));
#36194=CARTESIAN_POINT('Origin',(0.,0.,10.37));
#36195=CARTESIAN_POINT('Origin',(0.,0.,10.25));
#36196=CARTESIAN_POINT('',(-4.,-4.89858719658941E-16,10.13));
#36197=CARTESIAN_POINT('',(-4.,-4.89858719658941E-16,10.25));
#36198=CARTESIAN_POINT('',(4.,-4.89858719658941E-16,10.13));
#36199=CARTESIAN_POINT('Origin',(0.,0.,10.13));
#36200=CARTESIAN_POINT('Origin',(0.,0.,10.13));
#36201=CARTESIAN_POINT('Origin',(0.,0.,10.115));
#36202=CARTESIAN_POINT('',(3.985,4.8802174946022E-16,10.115));
#54965=UNCERTAINTY_MEASURE_WITH_UNIT(LENGTH_MEASURE(0.001),#55003,
'DISTANCE_ACCURACY_VALUE',
'Maximum model space distance between geometric entities at asserted c
onnectivities');
#54980=UNCERTAINTY_MEASURE_WITH_UNIT(LENGTH_MEASURE(0.001),#55003,
'DISTANCE_ACCURACY_VALUE',
'Maximum model space distance between geometric entities at asserted c
onnectivities');
#54987=(
GEOMETRIC_REPRESENTATION_CONTEXT(3)
GLOBAL_UNCERTAINTY_ASSIGNED_CONTEXT((#54965))
GLOBAL_UNIT_ASSIGNED_CONTEXT((#55003,#55005,#55006))
REPRESENTATION_CONTEXT('','3D')
);
#55002=(
GEOMETRIC_REPRESENTATION_CONTEXT(3)
GLOBAL_UNCERTAINTY_ASSIGNED_CONTEXT((#54980))
GLOBAL_UNIT_ASSIGNED_CONTEXT((#55003,#55005,#55006))
REPRESENTATION_CONTEXT('','3D')
);
#55003=(
LENGTH_UNIT()
NAMED_UNIT(*)
SI_UNIT(.CENTI.,.METRE.)
);
#55005=(
NAMED_UNIT(*)
PLANE_ANGLE_UNIT()
SI_UNIT($,.RADIAN.)
);
#55006=(
NAMED_UNIT(*)
SI_UNIT($,.STERADIAN.)
SOLID_ANGLE_UNIT()
);
#55013=SHAPE_DEFINITION_REPRESENTATION(#55034,#55109);
#55034=PRODUCT_DEFINITION_SHAPE('',$,#55131);
#55109=SHAPE_REPRESENTATION('',(#25749),#54987);
#55124=PRODUCT_DEFINITION_CONTEXT('part definition',#55189,'design');
#55131=PRODUCT_DEFINITION('2026-10-18-23-36-12-808',
'06_Motor_Mount_Bulkhead_Plate',#55152,#55124);
#55152=PRODUCT_DEFINITION_FORMATION('',$,#55197);
#55189=APPLICATION_CONTEXT(
'Core Data for Automotive Mechanical Design Process');
#55190=PRODUCT_CONTEXT('part definition',#55189,'mechanical');
#55197=PRODUCT('2026-10-18-23-36-12-808',
'06_Motor_Mount_Bulkhead_Plate',$,(#55190));
#55366=COLOUR_RGB('Light Blue',0.38,0.62,0.78);
#55367=FILL_AREA_STYLE_COLOUR('',#55366);
#55368=FILL_AREA_STYLE('',(#55367));
#55369=SURFACE_STYLE_FILL_AREA(#55368);
#55370=SURFACE_SIDE_STYLE('',(#55369));
#55371=SURFACE_STYLE_USAGE(.BOTH.,#55370);
#55372=PRESENTATION_STYLE_ASSIGNMENT((#55371));
ENDSEC;
END-ISO-10303-21;
